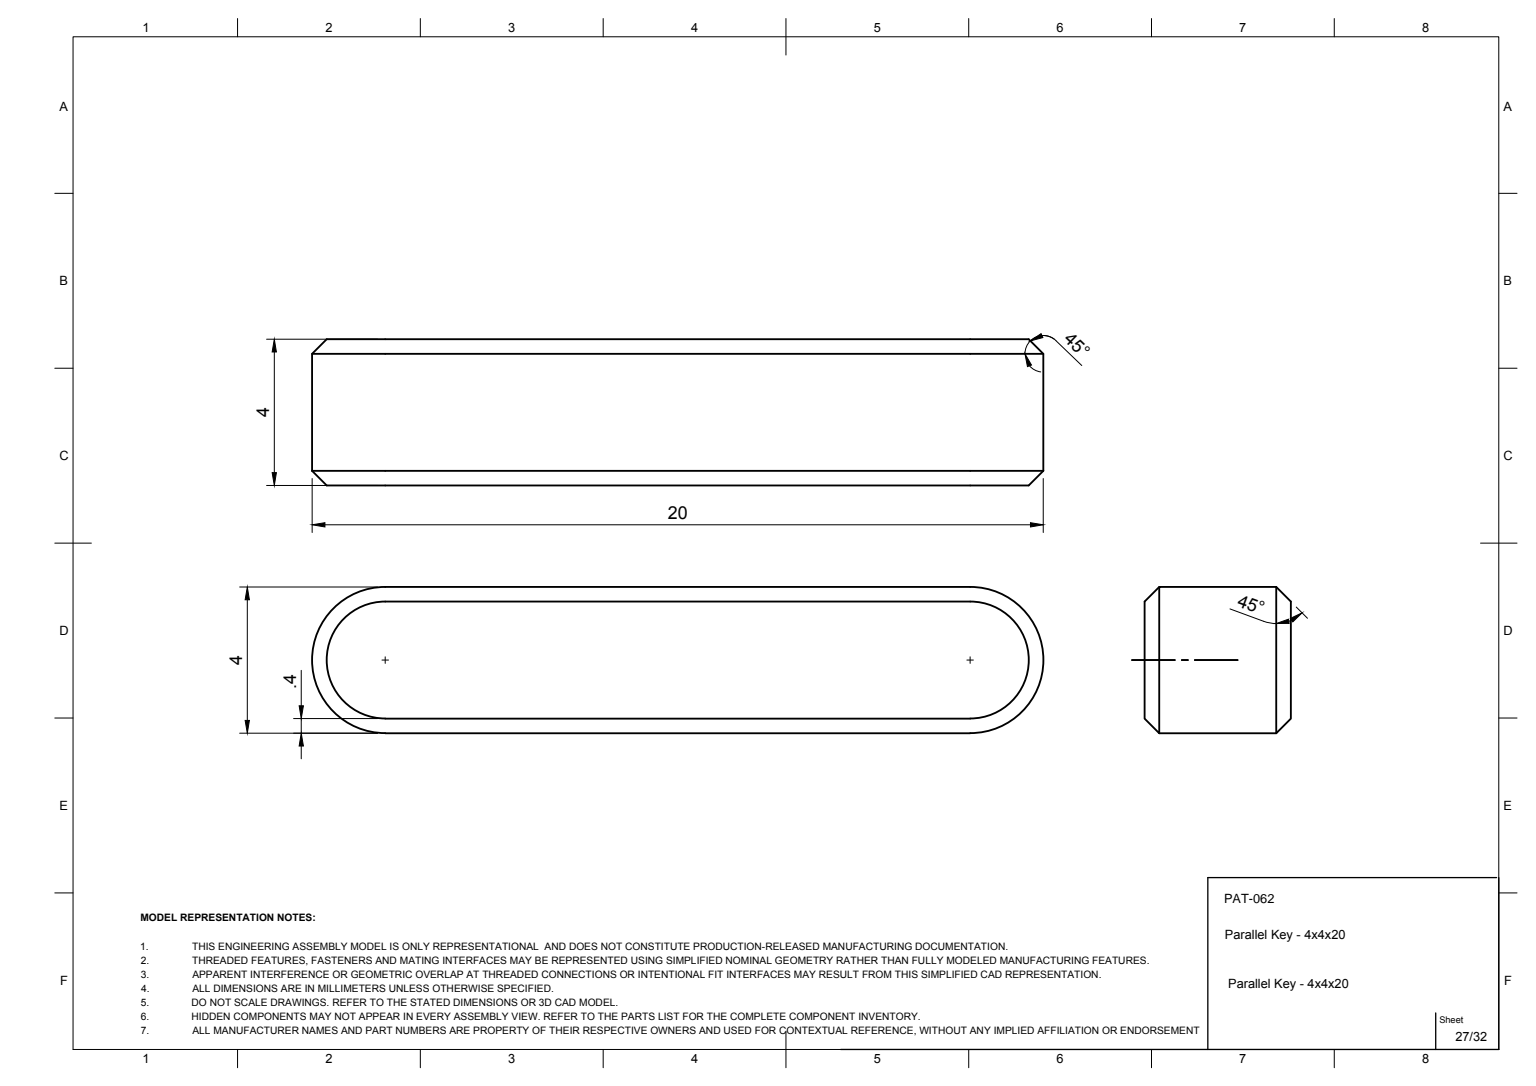
ISO-10303-21;
HEADER;
/* Generated by software containing ST-Developer
 * from STEP Tools, Inc. (www.steptools.com) 
 */

FILE_DESCRIPTION(
/* description */ ('Jaw-coupled motor to shaft test stand'),
/* implementation_level */ '2;1');

FILE_NAME(
/* name */ 'Parallel Key - 4x4x20.step',
/* time_stamp */ '2026-10-27T10:46:06-07:00',
/* author */ (''),
/* organization */ (''),
/* preprocessor_version */ 'ST-DEVELOPER v20.2',
/* originating_system */ 'Autodesk Translation Framework v15.17.0.0',
/* authorisation */ '');

FILE_SCHEMA (('AUTOMOTIVE_DESIGN { 1 0 10303 214 3 1 1 }'));
ENDSEC;

DATA;
#10=MECHANICAL_DESIGN_GEOMETRIC_PRESENTATION_REPRESENTATION('',(#370),#19361);
#19=CONICAL_SURFACE('',#12258,0.18,0.785398163397448);
#20=CONICAL_SURFACE('',#12262,0.18,0.785398163397448);
#21=CONICAL_SURFACE('',#12270,0.18,0.785398163397449);
#22=CONICAL_SURFACE('',#12273,0.18,0.785398163397449);
#305=SHAPE_REPRESENTATION_RELATIONSHIP('SRR','None',#19522,#337);
#337=ADVANCED_BREP_SHAPE_REPRESENTATION('',(#401),#19358);
#370=STYLED_ITEM('',(#19746),#401);
#401=MANIFOLD_SOLID_BREP('Body1',#11016);
#994=PLANE('',#12257);
#995=PLANE('',#12261);
#996=PLANE('',#12267);
#997=PLANE('',#12268);
#998=PLANE('',#12269);
#999=PLANE('',#12272);
#1000=PLANE('',#12277);
#1001=PLANE('',#12278);
#1599=FACE_OUTER_BOUND('',#2330,.T.);
#1600=FACE_OUTER_BOUND('',#2331,.T.);
#1601=FACE_OUTER_BOUND('',#2332,.T.);
#1602=FACE_OUTER_BOUND('',#2333,.T.);
#1603=FACE_OUTER_BOUND('',#2334,.T.);
#1604=FACE_OUTER_BOUND('',#2335,.T.);
#1605=FACE_OUTER_BOUND('',#2336,.T.);
#1606=FACE_OUTER_BOUND('',#2337,.T.);
#1607=FACE_OUTER_BOUND('',#2338,.T.);
#1608=FACE_OUTER_BOUND('',#2339,.T.);
#1609=FACE_OUTER_BOUND('',#2340,.T.);
#1610=FACE_OUTER_BOUND('',#2341,.T.);
#1611=FACE_OUTER_BOUND('',#2342,.T.);
#1612=FACE_OUTER_BOUND('',#2343,.T.);
#2330=EDGE_LOOP('',(#10100,#10101,#10102,#10103));
#2331=EDGE_LOOP('',(#10104,#10105,#10106,#10107));
#2332=EDGE_LOOP('',(#10108,#10109,#10110,#10111));
#2333=EDGE_LOOP('',(#10112,#10113,#10114,#10115));
#2334=EDGE_LOOP('',(#10116,#10117,#10118,#10119));
#2335=EDGE_LOOP('',(#10120,#10121,#10122,#10123));
#2336=EDGE_LOOP('',(#10124,#10125,#10126,#10127));
#2337=EDGE_LOOP('',(#10128,#10129,#10130,#10131));
#2338=EDGE_LOOP('',(#10132,#10133,#10134,#10135));
#2339=EDGE_LOOP('',(#10136,#10137,#10138,#10139));
#2340=EDGE_LOOP('',(#10140,#10141,#10142,#10143));
#2341=EDGE_LOOP('',(#10144,#10145,#10146,#10147));
#2342=EDGE_LOOP('',(#10148,#10149,#10150,#10151));
#2343=EDGE_LOOP('',(#10152,#10153,#10154,#10155));
#3463=LINE('',#19089,#4616);
#3464=LINE('',#19091,#4617);
#3465=LINE('',#19093,#4618);
#3466=LINE('',#19094,#4619);
#3467=LINE('',#19098,#4620);
#3468=LINE('',#19104,#4621);
#3469=LINE('',#19105,#4622);
#3470=LINE('',#19106,#4623);
#3471=LINE('',#19112,#4624);
#3472=LINE('',#19115,#4625);
#3473=LINE('',#19118,#4626);
#3474=LINE('',#19119,#4627);
#3475=LINE('',#19123,#4628);
#3476=LINE('',#19125,#4629);
#3477=LINE('',#19126,#4630);
#3478=LINE('',#19129,#4631);
#3479=LINE('',#19134,#4632);
#3480=LINE('',#19135,#4633);
#3481=LINE('',#19136,#4634);
#3482=LINE('',#19141,#4635);
#4616=VECTOR('',#15198,1.);
#4617=VECTOR('',#15199,1.);
#4618=VECTOR('',#15200,1.);
#4619=VECTOR('',#15201,1.);
#4620=VECTOR('',#15204,1.);
#4621=VECTOR('',#15211,1.);
#4622=VECTOR('',#15212,1.);
#4623=VECTOR('',#15213,1.);
#4624=VECTOR('',#15222,1.);
#4625=VECTOR('',#15225,1.);
#4626=VECTOR('',#15228,1.);
#4627=VECTOR('',#15229,1.);
#4628=VECTOR('',#15234,1.);
#4629=VECTOR('',#15235,1.);
#4630=VECTOR('',#15236,1.);
#4631=VECTOR('',#15239,1.);
#4632=VECTOR('',#15244,1.);
#4633=VECTOR('',#15245,1.);
#4634=VECTOR('',#15246,1.);
#4635=VECTOR('',#15255,1.);
#4923=CIRCLE('',#12259,0.16);
#4924=CIRCLE('',#12260,0.2);
#4925=CIRCLE('',#12263,0.16);
#4926=CIRCLE('',#12264,0.2);
#4927=CIRCLE('',#12266,0.2);
#4928=CIRCLE('',#12271,0.16);
#4929=CIRCLE('',#12274,0.2);
#4930=CIRCLE('',#12275,0.16);
#5832=VERTEX_POINT('',#19087);
#5833=VERTEX_POINT('',#19088);
#5834=VERTEX_POINT('',#19090);
#5835=VERTEX_POINT('',#19092);
#5836=VERTEX_POINT('',#19096);
#5837=VERTEX_POINT('',#19097);
#5838=VERTEX_POINT('',#19102);
#5839=VERTEX_POINT('',#19103);
#5840=VERTEX_POINT('',#19111);
#5841=VERTEX_POINT('',#19113);
#5842=VERTEX_POINT('',#19117);
#5843=VERTEX_POINT('',#19122);
#5844=VERTEX_POINT('',#19124);
#5845=VERTEX_POINT('',#19128);
#5846=VERTEX_POINT('',#19132);
#5847=VERTEX_POINT('',#19133);
#7261=EDGE_CURVE('',#5832,#5833,#3463,.T.);
#7262=EDGE_CURVE('',#5833,#5834,#3464,.T.);
#7263=EDGE_CURVE('',#5834,#5835,#3465,.T.);
#7264=EDGE_CURVE('',#5835,#5832,#3466,.T.);
#7265=EDGE_CURVE('',#5836,#5837,#3467,.T.);
#7266=EDGE_CURVE('',#5837,#5833,#4923,.T.);
#7267=EDGE_CURVE('',#5832,#5836,#4924,.T.);
#7268=EDGE_CURVE('',#5838,#5839,#3468,.T.);
#7269=EDGE_CURVE('',#5839,#5837,#3469,.T.);
#7270=EDGE_CURVE('',#5836,#5838,#3470,.T.);
#7271=EDGE_CURVE('',#5834,#5839,#4925,.T.);
#7272=EDGE_CURVE('',#5838,#5835,#4926,.T.);
#7273=EDGE_CURVE('',#5840,#5832,#3471,.T.);
#7274=EDGE_CURVE('',#5841,#5840,#4927,.T.);
#7275=EDGE_CURVE('',#5841,#5836,#3472,.T.);
#7276=EDGE_CURVE('',#5842,#5835,#3473,.T.);
#7277=EDGE_CURVE('',#5840,#5842,#3474,.T.);
#7278=EDGE_CURVE('',#5843,#5840,#3475,.T.);
#7279=EDGE_CURVE('',#5842,#5844,#3476,.T.);
#7280=EDGE_CURVE('',#5844,#5843,#3477,.T.);
#7281=EDGE_CURVE('',#5845,#5841,#3478,.T.);
#7282=EDGE_CURVE('',#5843,#5845,#4928,.T.);
#7283=EDGE_CURVE('',#5846,#5847,#3479,.T.);
#7284=EDGE_CURVE('',#5847,#5841,#3480,.T.);
#7285=EDGE_CURVE('',#5845,#5846,#3481,.T.);
#7286=EDGE_CURVE('',#5842,#5847,#4929,.T.);
#7287=EDGE_CURVE('',#5846,#5844,#4930,.T.);
#7288=EDGE_CURVE('',#5847,#5838,#3482,.T.);
#10100=ORIENTED_EDGE('',*,*,#7261,.T.);
#10101=ORIENTED_EDGE('',*,*,#7262,.T.);
#10102=ORIENTED_EDGE('',*,*,#7263,.T.);
#10103=ORIENTED_EDGE('',*,*,#7264,.T.);
#10104=ORIENTED_EDGE('',*,*,#7265,.T.);
#10105=ORIENTED_EDGE('',*,*,#7266,.T.);
#10106=ORIENTED_EDGE('',*,*,#7261,.F.);
#10107=ORIENTED_EDGE('',*,*,#7267,.T.);
#10108=ORIENTED_EDGE('',*,*,#7268,.T.);
#10109=ORIENTED_EDGE('',*,*,#7269,.T.);
#10110=ORIENTED_EDGE('',*,*,#7265,.F.);
#10111=ORIENTED_EDGE('',*,*,#7270,.T.);
#10112=ORIENTED_EDGE('',*,*,#7263,.F.);
#10113=ORIENTED_EDGE('',*,*,#7271,.T.);
#10114=ORIENTED_EDGE('',*,*,#7268,.F.);
#10115=ORIENTED_EDGE('',*,*,#7272,.T.);
#10116=ORIENTED_EDGE('',*,*,#7267,.F.);
#10117=ORIENTED_EDGE('',*,*,#7273,.F.);
#10118=ORIENTED_EDGE('',*,*,#7274,.F.);
#10119=ORIENTED_EDGE('',*,*,#7275,.T.);
#10120=ORIENTED_EDGE('',*,*,#7264,.F.);
#10121=ORIENTED_EDGE('',*,*,#7276,.F.);
#10122=ORIENTED_EDGE('',*,*,#7277,.F.);
#10123=ORIENTED_EDGE('',*,*,#7273,.T.);
#10124=ORIENTED_EDGE('',*,*,#7262,.F.);
#10125=ORIENTED_EDGE('',*,*,#7266,.F.);
#10126=ORIENTED_EDGE('',*,*,#7269,.F.);
#10127=ORIENTED_EDGE('',*,*,#7271,.F.);
#10128=ORIENTED_EDGE('',*,*,#7278,.T.);
#10129=ORIENTED_EDGE('',*,*,#7277,.T.);
#10130=ORIENTED_EDGE('',*,*,#7279,.T.);
#10131=ORIENTED_EDGE('',*,*,#7280,.T.);
#10132=ORIENTED_EDGE('',*,*,#7281,.T.);
#10133=ORIENTED_EDGE('',*,*,#7274,.T.);
#10134=ORIENTED_EDGE('',*,*,#7278,.F.);
#10135=ORIENTED_EDGE('',*,*,#7282,.T.);
#10136=ORIENTED_EDGE('',*,*,#7283,.T.);
#10137=ORIENTED_EDGE('',*,*,#7284,.T.);
#10138=ORIENTED_EDGE('',*,*,#7281,.F.);
#10139=ORIENTED_EDGE('',*,*,#7285,.T.);
#10140=ORIENTED_EDGE('',*,*,#7279,.F.);
#10141=ORIENTED_EDGE('',*,*,#7286,.T.);
#10142=ORIENTED_EDGE('',*,*,#7283,.F.);
#10143=ORIENTED_EDGE('',*,*,#7287,.T.);
#10144=ORIENTED_EDGE('',*,*,#7272,.F.);
#10145=ORIENTED_EDGE('',*,*,#7288,.F.);
#10146=ORIENTED_EDGE('',*,*,#7286,.F.);
#10147=ORIENTED_EDGE('',*,*,#7276,.T.);
#10148=ORIENTED_EDGE('',*,*,#7280,.F.);
#10149=ORIENTED_EDGE('',*,*,#7287,.F.);
#10150=ORIENTED_EDGE('',*,*,#7285,.F.);
#10151=ORIENTED_EDGE('',*,*,#7282,.F.);
#10152=ORIENTED_EDGE('',*,*,#7270,.F.);
#10153=ORIENTED_EDGE('',*,*,#7275,.F.);
#10154=ORIENTED_EDGE('',*,*,#7284,.F.);
#10155=ORIENTED_EDGE('',*,*,#7288,.T.);
#10359=CYLINDRICAL_SURFACE('',#12265,0.2);
#10360=CYLINDRICAL_SURFACE('',#12276,0.2);
#10941=ADVANCED_FACE('',(#1599),#994,.T.);
#10942=ADVANCED_FACE('',(#1600),#19,.T.);
#10943=ADVANCED_FACE('',(#1601),#995,.T.);
#10944=ADVANCED_FACE('',(#1602),#20,.T.);
#10945=ADVANCED_FACE('',(#1603),#10359,.T.);
#10946=ADVANCED_FACE('',(#1604),#996,.T.);
#10947=ADVANCED_FACE('',(#1605),#997,.T.);
#10948=ADVANCED_FACE('',(#1606),#998,.T.);
#10949=ADVANCED_FACE('',(#1607),#21,.T.);
#10950=ADVANCED_FACE('',(#1608),#999,.T.);
#10951=ADVANCED_FACE('',(#1609),#22,.T.);
#10952=ADVANCED_FACE('',(#1610),#10360,.T.);
#10953=ADVANCED_FACE('',(#1611),#1000,.F.);
#10954=ADVANCED_FACE('',(#1612),#1001,.T.);
#11016=CLOSED_SHELL('',(#10941,#10942,#10943,#10944,#10945,#10946,#10947,
#10948,#10949,#10950,#10951,#10952,#10953,#10954));
#12256=AXIS2_PLACEMENT_3D('',#19085,#15194,#15195);
#12257=AXIS2_PLACEMENT_3D('',#19086,#15196,#15197);
#12258=AXIS2_PLACEMENT_3D('',#19095,#15202,#15203);
#12259=AXIS2_PLACEMENT_3D('',#19099,#15205,#15206);
#12260=AXIS2_PLACEMENT_3D('',#19100,#15207,#15208);
#12261=AXIS2_PLACEMENT_3D('',#19101,#15209,#15210);
#12262=AXIS2_PLACEMENT_3D('',#19107,#15214,#15215);
#12263=AXIS2_PLACEMENT_3D('',#19108,#15216,#15217);
#12264=AXIS2_PLACEMENT_3D('',#19109,#15218,#15219);
#12265=AXIS2_PLACEMENT_3D('',#19110,#15220,#15221);
#12266=AXIS2_PLACEMENT_3D('',#19114,#15223,#15224);
#12267=AXIS2_PLACEMENT_3D('',#19116,#15226,#15227);
#12268=AXIS2_PLACEMENT_3D('',#19120,#15230,#15231);
#12269=AXIS2_PLACEMENT_3D('',#19121,#15232,#15233);
#12270=AXIS2_PLACEMENT_3D('',#19127,#15237,#15238);
#12271=AXIS2_PLACEMENT_3D('',#19130,#15240,#15241);
#12272=AXIS2_PLACEMENT_3D('',#19131,#15242,#15243);
#12273=AXIS2_PLACEMENT_3D('',#19137,#15247,#15248);
#12274=AXIS2_PLACEMENT_3D('',#19138,#15249,#15250);
#12275=AXIS2_PLACEMENT_3D('',#19139,#15251,#15252);
#12276=AXIS2_PLACEMENT_3D('',#19140,#15253,#15254);
#12277=AXIS2_PLACEMENT_3D('',#19142,#15256,#15257);
#12278=AXIS2_PLACEMENT_3D('',#19143,#15258,#15259);
#15194=DIRECTION('axis',(0.,0.,1.));
#15195=DIRECTION('refdir',(1.,0.,0.));
#15196=DIRECTION('center_axis',(0.,0.707106781186548,0.707106781186547));
#15197=DIRECTION('ref_axis',(1.,0.,0.));
#15198=DIRECTION('',(-1.96261557335472E-15,-0.707106781186547,0.707106781186548));
#15199=DIRECTION('',(1.,0.,0.));
#15200=DIRECTION('',(0.,0.707106781186547,-0.707106781186548));
#15201=DIRECTION('',(-1.,0.,0.));
#15202=DIRECTION('center_axis',(0.,0.,-1.));
#15203=DIRECTION('ref_axis',(0.,1.,0.));
#15204=DIRECTION('',(0.,0.707106781186548,0.707106781186548));
#15205=DIRECTION('center_axis',(0.,0.,-1.));
#15206=DIRECTION('ref_axis',(0.,1.,0.));
#15207=DIRECTION('center_axis',(0.,0.,1.));
#15208=DIRECTION('ref_axis',(0.,1.,0.));
#15209=DIRECTION('center_axis',(0.,-0.707106781186548,0.707106781186547));
#15210=DIRECTION('ref_axis',(1.,0.,0.));
#15211=DIRECTION('',(1.96261557335472E-15,0.707106781186547,0.707106781186548));
#15212=DIRECTION('',(-1.,0.,0.));
#15213=DIRECTION('',(1.,0.,0.));
#15214=DIRECTION('center_axis',(0.,0.,-1.));
#15215=DIRECTION('ref_axis',(0.,-1.,0.));
#15216=DIRECTION('center_axis',(0.,0.,-1.));
#15217=DIRECTION('ref_axis',(0.,-1.,0.));
#15218=DIRECTION('center_axis',(0.,0.,1.));
#15219=DIRECTION('ref_axis',(0.,-1.,0.));
#15220=DIRECTION('center_axis',(0.,0.,1.));
#15221=DIRECTION('ref_axis',(0.,1.,0.));
#15222=DIRECTION('',(0.,0.,1.));
#15223=DIRECTION('center_axis',(0.,0.,-1.));
#15224=DIRECTION('ref_axis',(0.,1.,0.));
#15225=DIRECTION('',(0.,0.,1.));
#15226=DIRECTION('center_axis',(0.,1.,0.));
#15227=DIRECTION('ref_axis',(-1.,0.,0.));
#15228=DIRECTION('',(0.,0.,1.));
#15229=DIRECTION('',(1.,0.,0.));
#15230=DIRECTION('center_axis',(0.,0.,1.));
#15231=DIRECTION('ref_axis',(1.,0.,0.));
#15232=DIRECTION('center_axis',(0.,0.707106781186548,-0.707106781186548));
#15233=DIRECTION('ref_axis',(-1.,0.,0.));
#15234=DIRECTION('',(1.96261557335472E-15,0.707106781186548,0.707106781186548));
#15235=DIRECTION('',(0.,-0.707106781186548,-0.707106781186548));
#15236=DIRECTION('',(-1.,0.,0.));
#15237=DIRECTION('center_axis',(0.,0.,1.));
#15238=DIRECTION('ref_axis',(0.,1.,0.));
#15239=DIRECTION('',(0.,-0.707106781186548,0.707106781186547));
#15240=DIRECTION('center_axis',(0.,0.,1.));
#15241=DIRECTION('ref_axis',(0.,1.,0.));
#15242=DIRECTION('center_axis',(0.,-0.707106781186548,-0.707106781186548));
#15243=DIRECTION('ref_axis',(-1.,0.,0.));
#15244=DIRECTION('',(-1.96261557335472E-15,-0.707106781186548,0.707106781186548));
#15245=DIRECTION('',(-1.,0.,0.));
#15246=DIRECTION('',(1.,0.,0.));
#15247=DIRECTION('center_axis',(0.,0.,1.));
#15248=DIRECTION('ref_axis',(0.,-1.,0.));
#15249=DIRECTION('center_axis',(0.,0.,-1.));
#15250=DIRECTION('ref_axis',(0.,-1.,0.));
#15251=DIRECTION('center_axis',(0.,0.,1.));
#15252=DIRECTION('ref_axis',(0.,-1.,0.));
#15253=DIRECTION('center_axis',(0.,0.,1.));
#15254=DIRECTION('ref_axis',(0.,-1.,0.));
#15255=DIRECTION('',(0.,0.,1.));
#15256=DIRECTION('center_axis',(0.,0.,1.));
#15257=DIRECTION('ref_axis',(1.,0.,0.));
#15258=DIRECTION('center_axis',(0.,-1.,0.));
#15259=DIRECTION('ref_axis',(1.,0.,0.));
#19085=CARTESIAN_POINT('',(0.,0.,0.));
#19086=CARTESIAN_POINT('Origin',(0.4,0.18,0.38));
#19087=CARTESIAN_POINT('',(-0.8,0.2,0.36));
#19088=CARTESIAN_POINT('',(-0.8,0.16,0.4));
#19089=CARTESIAN_POINT('',(-0.8,0.2,0.36));
#19090=CARTESIAN_POINT('',(0.8,0.16,0.4));
#19091=CARTESIAN_POINT('',(0.4,0.16,0.4));
#19092=CARTESIAN_POINT('',(0.8,0.2,0.36));
#19093=CARTESIAN_POINT('',(0.8,0.16,0.4));
#19094=CARTESIAN_POINT('',(0.4,0.2,0.36));
#19095=CARTESIAN_POINT('Origin',(-0.8,0.,0.38));
#19096=CARTESIAN_POINT('',(-0.8,-0.2,0.36));
#19097=CARTESIAN_POINT('',(-0.8,-0.16,0.4));
#19098=CARTESIAN_POINT('',(-0.8,-0.2,0.36));
#19099=CARTESIAN_POINT('Origin',(-0.8,0.,0.4));
#19100=CARTESIAN_POINT('Origin',(-0.8,0.,0.36));
#19101=CARTESIAN_POINT('Origin',(-0.4,-0.18,0.38));
#19102=CARTESIAN_POINT('',(0.8,-0.2,0.36));
#19103=CARTESIAN_POINT('',(0.8,-0.16,0.4));
#19104=CARTESIAN_POINT('',(0.8,-0.2,0.36));
#19105=CARTESIAN_POINT('',(-0.4,-0.16,0.4));
#19106=CARTESIAN_POINT('',(-0.4,-0.2,0.36));
#19107=CARTESIAN_POINT('Origin',(0.8,0.,0.38));
#19108=CARTESIAN_POINT('Origin',(0.8,0.,0.4));
#19109=CARTESIAN_POINT('Origin',(0.8,0.,0.36));
#19110=CARTESIAN_POINT('Origin',(-0.8,0.,0.));
#19111=CARTESIAN_POINT('',(-0.8,0.2,0.04));
#19112=CARTESIAN_POINT('',(-0.8,0.2,0.));
#19113=CARTESIAN_POINT('',(-0.8,-0.2,0.04));
#19114=CARTESIAN_POINT('Origin',(-0.8,0.,0.04));
#19115=CARTESIAN_POINT('',(-0.8,-0.2,0.));
#19116=CARTESIAN_POINT('Origin',(0.8,0.2,0.));
#19117=CARTESIAN_POINT('',(0.8,0.2,0.04));
#19118=CARTESIAN_POINT('',(0.8,0.2,0.));
#19119=CARTESIAN_POINT('',(0.4,0.2,0.04));
#19120=CARTESIAN_POINT('Origin',(0.,0.,0.4));
#19121=CARTESIAN_POINT('Origin',(0.4,0.18,0.02));
#19122=CARTESIAN_POINT('',(-0.8,0.16,0.));
#19123=CARTESIAN_POINT('',(-0.8,0.16,0.));
#19124=CARTESIAN_POINT('',(0.8,0.16,0.));
#19125=CARTESIAN_POINT('',(0.8,0.2,0.04));
#19126=CARTESIAN_POINT('',(0.4,0.16,0.));
#19127=CARTESIAN_POINT('Origin',(-0.8,0.,0.02));
#19128=CARTESIAN_POINT('',(-0.8,-0.16,0.));
#19129=CARTESIAN_POINT('',(-0.8,-0.16,0.));
#19130=CARTESIAN_POINT('Origin',(-0.8,0.,0.));
#19131=CARTESIAN_POINT('Origin',(-0.4,-0.18,0.02));
#19132=CARTESIAN_POINT('',(0.8,-0.16,0.));
#19133=CARTESIAN_POINT('',(0.8,-0.2,0.04));
#19134=CARTESIAN_POINT('',(0.8,-0.16,0.));
#19135=CARTESIAN_POINT('',(-0.4,-0.2,0.04));
#19136=CARTESIAN_POINT('',(-0.4,-0.16,0.));
#19137=CARTESIAN_POINT('Origin',(0.8,0.,0.02));
#19138=CARTESIAN_POINT('Origin',(0.8,0.,0.04));
#19139=CARTESIAN_POINT('Origin',(0.8,0.,0.));
#19140=CARTESIAN_POINT('Origin',(0.8,0.,0.));
#19141=CARTESIAN_POINT('',(0.8,-0.2,0.));
#19142=CARTESIAN_POINT('Origin',(0.,0.,0.));
#19143=CARTESIAN_POINT('Origin',(-0.8,-0.2,0.));
#19320=UNCERTAINTY_MEASURE_WITH_UNIT(LENGTH_MEASURE(0.001),#19362,
'DISTANCE_ACCURACY_VALUE',
'Maximum model space distance between geometric entities at asserted c
onnectivities');
#19323=UNCERTAINTY_MEASURE_WITH_UNIT(LENGTH_MEASURE(0.001),#19362,
'DISTANCE_ACCURACY_VALUE',
'Maximum model space distance between geometric entities at asserted c
onnectivities');
#19358=(
GEOMETRIC_REPRESENTATION_CONTEXT(3)
GLOBAL_UNCERTAINTY_ASSIGNED_CONTEXT((#19320))
GLOBAL_UNIT_ASSIGNED_CONTEXT((#19362,#19364,#19365))
REPRESENTATION_CONTEXT('','3D')
);
#19361=(
GEOMETRIC_REPRESENTATION_CONTEXT(3)
GLOBAL_UNCERTAINTY_ASSIGNED_CONTEXT((#19323))
GLOBAL_UNIT_ASSIGNED_CONTEXT((#19362,#19364,#19365))
REPRESENTATION_CONTEXT('','3D')
);
#19362=(
LENGTH_UNIT()
NAMED_UNIT(*)
SI_UNIT(.CENTI.,.METRE.)
);
#19364=(
NAMED_UNIT(*)
PLANE_ANGLE_UNIT()
SI_UNIT($,.RADIAN.)
);
#19365=(
NAMED_UNIT(*)
SI_UNIT($,.STERADIAN.)
SOLID_ANGLE_UNIT()
);
#19400=SHAPE_DEFINITION_REPRESENTATION(#19467,#19522);
#19467=PRODUCT_DEFINITION_SHAPE('',$,#19560);
#19522=SHAPE_REPRESENTATION('',(#12256),#19358);
#19525=PRODUCT_DEFINITION_CONTEXT('part definition',#19638,'design');
#19560=PRODUCT_DEFINITION('Parallel Key - 4x4x20',
'Parallel Key - 4x4x20',#19597,#19525);
#19597=PRODUCT_DEFINITION_FORMATION('',$,#19674);
#19638=APPLICATION_CONTEXT(
'Core Data for Automotive Mechanical Design Process');
#19639=PRODUCT_CONTEXT('part definition',#19638,'mechanical');
#19674=PRODUCT('Parallel Key - 4x4x20','Parallel Key - 4x4x20',
'Parallel Key - 4x4x20',(#19639));
#19740=COLOUR_RGB('Grey',0.48,0.52,0.57);
#19741=FILL_AREA_STYLE_COLOUR('',#19740);
#19742=FILL_AREA_STYLE('',(#19741));
#19743=SURFACE_STYLE_FILL_AREA(#19742);
#19744=SURFACE_SIDE_STYLE('',(#19743));
#19745=SURFACE_STYLE_USAGE(.BOTH.,#19744);
#19746=PRESENTATION_STYLE_ASSIGNMENT((#19745));
ENDSEC;
END-ISO-10303-21;
